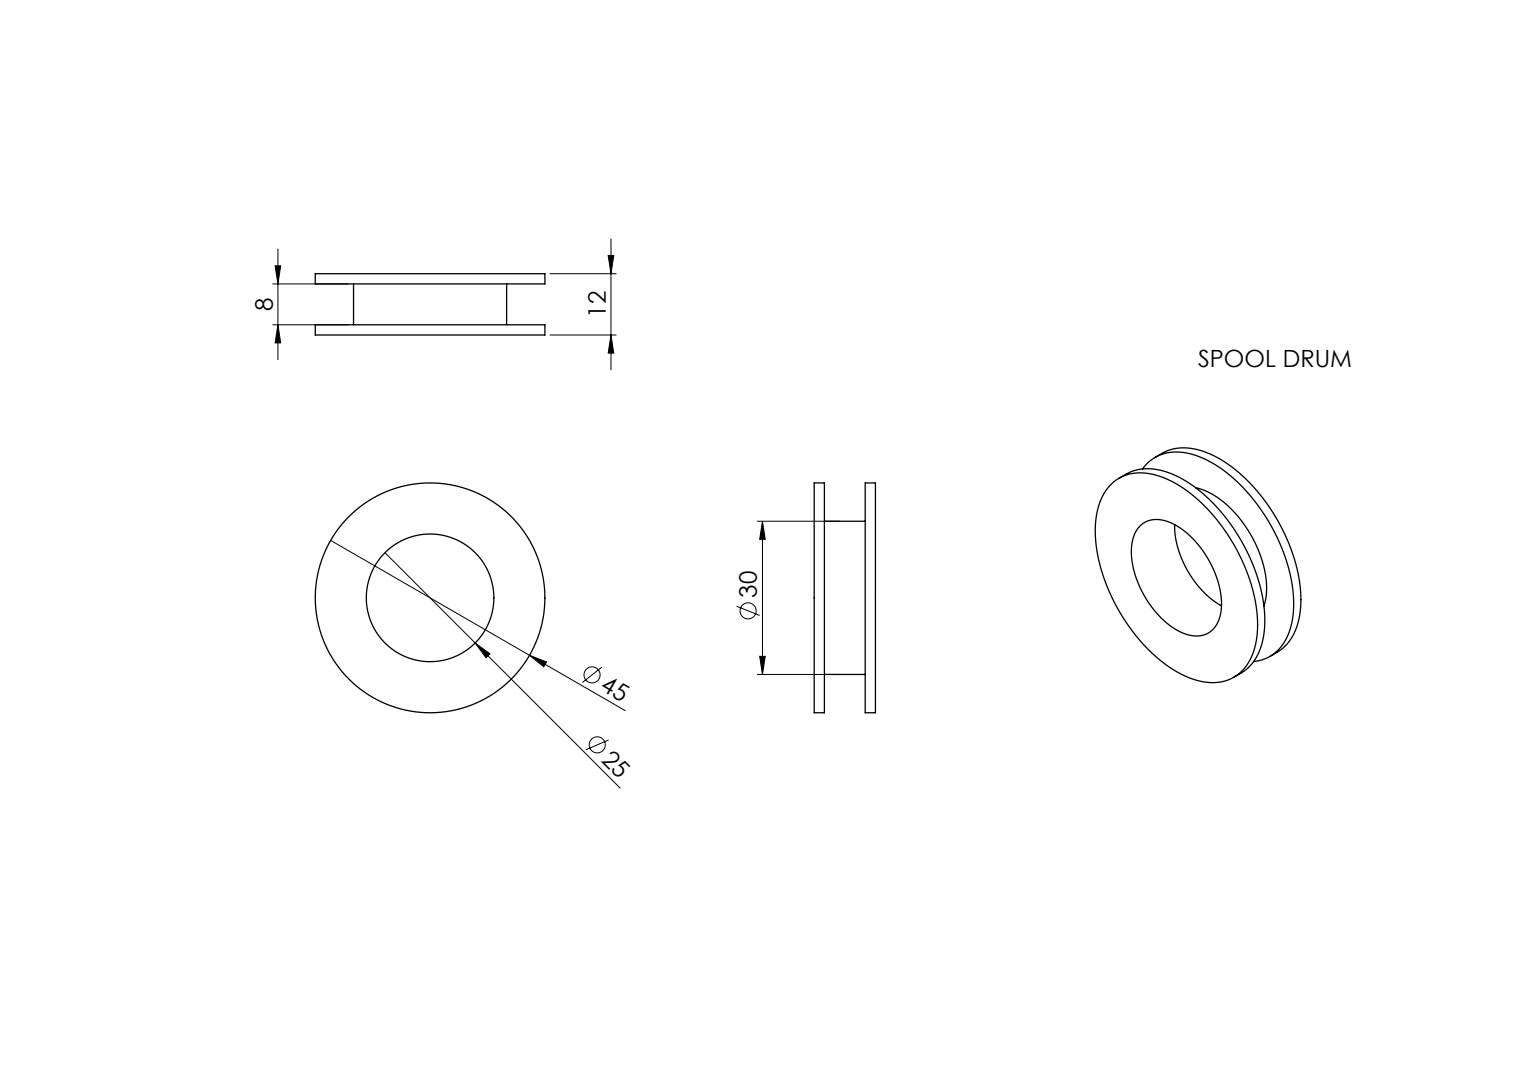
ISO-10303-21;
HEADER;
FILE_DESCRIPTION (('STEP AP214'),
    '1' );
FILE_NAME ('Spool Drum.step',
    '2026-10-23T14:45:25',
    ( '' ),
    ( '' ),
    'SwSTEP 2.0',
    'SolidWorks 2026',
    '' );
FILE_SCHEMA (( 'AUTOMOTIVE_DESIGN' ));
ENDSEC;

DATA;
#15=FACE_OUTER_BOUND ( 'NONE', #2318, .T. ) ;
#31=DIRECTION ( 'NONE',  ( -1.000000000000000000, 0.000000000000000000, 0.000000000000000000 ) ) ;
#54=VECTOR ( 'NONE', #1585, 1000.000000000000000 ) ;
#63=CARTESIAN_POINT ( 'NONE',  ( -12.50000000000000000, 0.000000000000000000, 14.00000000000000000 ) ) ;
#87=DIRECTION ( 'NONE',  ( 0.000000000000000000, 0.000000000000000000, -1.000000000000000000 ) ) ;
#91=DIRECTION ( 'NONE',  ( -0.000000000000000000, -0.000000000000000000, -1.000000000000000000 ) ) ;
#105=EDGE_CURVE ( 'NONE', #3518, #3244, #4364, .T. ) ;
#128=CARTESIAN_POINT ( 'NONE',  ( 22.50000000000000355, 2.755455298081545172E-15, 4.000000000000000000 ) ) ;
#145=LINE ( 'NONE', #1902, #3817 ) ;
#163=CIRCLE ( 'NONE', #2186, 15.00000000000000000 ) ;
#167=EDGE_CURVE ( 'NONE', #3046, #5218, #4525, .T. ) ;
#199=CARTESIAN_POINT ( 'NONE',  ( 0.000000000000000000, 0.000000000000000000, 12.00000000000000000 ) ) ;
#201=CARTESIAN_POINT ( 'NONE',  ( 0.000000000000000000, 0.000000000000000000, 14.00000000000000000 ) ) ;
#271=EDGE_LOOP ( 'NONE', ( #2578, #2682 ) ) ;
#283=CARTESIAN_POINT ( 'NONE',  ( 0.000000000000000000, 0.000000000000000000, 0.000000000000000000 ) ) ;
#310=( LENGTH_UNIT ( ) NAMED_UNIT ( * ) SI_UNIT ( .MILLI., .METRE. ) );
#312=ADVANCED_FACE ( 'NONE', ( #3377 ), #4350, .T. ) ;
#318=AXIS2_PLACEMENT_3D ( 'NONE', #1588, #1158, #4183 ) ;
#328=EDGE_CURVE ( 'NONE', #3244, #3518, #3734, .T. ) ;
#336=CARTESIAN_POINT ( 'NONE',  ( 0.000000000000000000, 0.000000000000000000, 4.000000000000000000 ) ) ;
#388=FACE_OUTER_BOUND ( 'NONE', #4673, .T. ) ;
#404=DIRECTION ( 'NONE',  ( 0.000000000000000000, 0.000000000000000000, 1.000000000000000000 ) ) ;
#409=PRODUCT_DEFINITION_SHAPE ( 'NONE', 'NONE',  #1447 ) ;
#414=AXIS2_PLACEMENT_3D ( 'NONE', #201, #3683, #2416 ) ;
#420=ORIENTED_EDGE ( 'NONE', *, *, #5372, .T. ) ;
#436=ORIENTED_EDGE ( 'NONE', *, *, #1530, .T. ) ;
#464=CARTESIAN_POINT ( 'NONE',  ( 0.000000000000000000, 0.000000000000000000, 14.00000000000000000 ) ) ;
#473=CARTESIAN_POINT ( 'NONE',  ( 0.000000000000000000, 0.000000000000000000, 2.000000000000000000 ) ) ;
#479=DIRECTION ( 'NONE',  ( 1.000000000000000000, 0.000000000000000000, 0.000000000000000000 ) ) ;
#484=DIRECTION ( 'NONE',  ( 0.000000000000000000, 0.000000000000000000, -1.000000000000000000 ) ) ;
#499=AXIS2_PLACEMENT_3D ( 'NONE', #336, #5518, #5170 ) ;
#520=AXIS2_PLACEMENT_3D ( 'NONE', #3033, #5131, #3456 ) ;
#534=VERTEX_POINT ( 'NONE', #2654 ) ;
#551=ORIENTED_EDGE ( 'NONE', *, *, #167, .T. ) ;
#567=ORIENTED_EDGE ( 'NONE', *, *, #695, .F. ) ;
#585=EDGE_CURVE ( 'NONE', #2034, #5308, #1351, .T. ) ;
#618=ORIENTED_EDGE ( 'NONE', *, *, #1353, .F. ) ;
#625=AXIS2_PLACEMENT_3D ( 'NONE', #1558, #3738, #1899 ) ;
#627=ORIENTED_EDGE ( 'NONE', *, *, #328, .T. ) ;
#647=DIRECTION ( 'NONE',  ( -0.000000000000000000, -0.000000000000000000, -1.000000000000000000 ) ) ;
#665=UNCERTAINTY_MEASURE_WITH_UNIT (LENGTH_MEASURE( 1.000000000000000082E-05 ), #5331, 'distance_accuracy_value', 'NONE');
#667=ORIENTED_EDGE ( 'NONE', *, *, #1697, .T. ) ;
#673=EDGE_LOOP ( 'NONE', ( #3634, #1342, #551, #4466 ) ) ;
#695=EDGE_CURVE ( 'NONE', #5417, #2009, #2414, .T. ) ;
#702=CARTESIAN_POINT ( 'NONE',  ( -22.50000000000000355, 0.000000000000000000, 14.00000000000000000 ) ) ;
#732=ORIENTED_EDGE ( 'NONE', *, *, #5425, .T. ) ;
#775=ADVANCED_FACE ( 'NONE', ( #4519, #5412 ), #2791, .T. ) ;
#781=DIRECTION ( 'NONE',  ( 1.000000000000000000, 0.000000000000000000, 0.000000000000000000 ) ) ;
#785=AXIS2_PLACEMENT_3D ( 'NONE', #3064, #2598, #871 ) ;
#801=DIRECTION ( 'NONE',  ( -1.000000000000000000, 0.000000000000000000, 0.000000000000000000 ) ) ;
#811=ORIENTED_EDGE ( 'NONE', *, *, #5425, .F. ) ;
#834=( NAMED_UNIT ( * ) SI_UNIT ( $, .STERADIAN. ) SOLID_ANGLE_UNIT ( ) );
#859=CIRCLE ( 'NONE', #4991, 12.50000000000000000 ) ;
#863=CIRCLE ( 'NONE', #5184, 22.50000000000000355 ) ;
#871=DIRECTION ( 'NONE',  ( -1.000000000000000000, 0.000000000000000000, 0.000000000000000000 ) ) ;
#881=CARTESIAN_POINT ( 'NONE',  ( -22.50000000000000355, 0.000000000000000000, 2.000000000000000000 ) ) ;
#886=AXIS2_PLACEMENT_3D ( 'NONE', #464, #4037, #4065 ) ;
#900=DIRECTION ( 'NONE',  ( -1.000000000000000000, 0.000000000000000000, 0.000000000000000000 ) ) ;
#934=ORIENTED_EDGE ( 'NONE', *, *, #585, .F. ) ;
#936=PLANE ( 'NONE',  #4756 ) ;
#1043=FACE_OUTER_BOUND ( 'NONE', #2938, .T. ) ;
#1046=CIRCLE ( 'NONE', #1974, 15.00000000000000000 ) ;
#1062=CARTESIAN_POINT ( 'NONE',  ( -22.50000000000000355, 0.000000000000000000, 14.00000000000000000 ) ) ;
#1091=DIRECTION ( 'NONE',  ( 0.000000000000000000, 0.000000000000000000, -1.000000000000000000 ) ) ;
#1117=VERTEX_POINT ( 'NONE', #1252 ) ;
#1119=DIRECTION ( 'NONE',  ( -1.000000000000000000, 0.000000000000000000, 0.000000000000000000 ) ) ;
#1131=DIRECTION ( 'NONE',  ( -1.000000000000000000, 0.000000000000000000, 0.000000000000000000 ) ) ;
#1158=DIRECTION ( 'NONE',  ( 0.000000000000000000, 0.000000000000000000, -1.000000000000000000 ) ) ;
#1172=AXIS2_PLACEMENT_3D ( 'NONE', #4145, #1091, #3312 ) ;
#1178=DIRECTION ( 'NONE',  ( 0.000000000000000000, 0.000000000000000000, -1.000000000000000000 ) ) ;
#1183=( NAMED_UNIT ( * ) PLANE_ANGLE_UNIT ( ) SI_UNIT ( $, .RADIAN. ) );
#1195=PRODUCT ( 'Spool Drum', 'Spool Drum', '', ( #4370 ) ) ;
#1196=CYLINDRICAL_SURFACE ( 'NONE', #785, 22.50000000000000355 ) ;
#1223=ORIENTED_EDGE ( 'NONE', *, *, #3217, .T. ) ;
#1230=DIRECTION ( 'NONE',  ( -0.000000000000000000, -0.000000000000000000, -1.000000000000000000 ) ) ;
#1247=AXIS2_PLACEMENT_3D ( 'NONE', #1760, #1390, #900 ) ;
#1252=CARTESIAN_POINT ( 'NONE',  ( -12.50000000000000000, 0.000000000000000000, 2.000000000000000000 ) ) ;
#1267=DIRECTION ( 'NONE',  ( 0.000000000000000000, 0.000000000000000000, 1.000000000000000000 ) ) ;
#1273=ORIENTED_EDGE ( 'NONE', *, *, #3459, .T. ) ;
#1276=CARTESIAN_POINT ( 'NONE',  ( 0.000000000000000000, 0.000000000000000000, 2.000000000000000000 ) ) ;
#1295=EDGE_CURVE ( 'NONE', #1815, #3046, #2550, .T. ) ;
#1301=DIRECTION ( 'NONE',  ( -1.000000000000000000, 0.000000000000000000, 0.000000000000000000 ) ) ;
#1336=AXIS2_PLACEMENT_3D ( 'NONE', #283, #2997, #5213 ) ;
#1342=ORIENTED_EDGE ( 'NONE', *, *, #4524, .F. ) ;
#1351=CIRCLE ( 'NONE', #4561, 15.00000000000000000 ) ;
#1353=EDGE_CURVE ( 'NONE', #4627, #4235, #163, .T. ) ;
#1355=DIRECTION ( 'NONE',  ( -0.000000000000000000, -0.000000000000000000, -1.000000000000000000 ) ) ;
#1367=ORIENTED_EDGE ( 'NONE', *, *, #5002, .T. ) ;
#1383=CARTESIAN_POINT ( 'NONE',  ( 0.000000000000000000, 0.000000000000000000, 12.00000000000000000 ) ) ;
#1390=DIRECTION ( 'NONE',  ( 0.000000000000000000, 0.000000000000000000, -1.000000000000000000 ) ) ;
#1414=( NAMED_UNIT ( * ) SI_UNIT ( $, .STERADIAN. ) SOLID_ANGLE_UNIT ( ) );
#1427=CARTESIAN_POINT ( 'NONE',  ( 15.00000000000000000, 1.836970198721029589E-15, 4.000000000000000000 ) ) ;
#1447=PRODUCT_DEFINITION ( 'UNKNOWN', '', #5080, #1714 ) ;
#1485=ORIENTED_EDGE ( 'NONE', *, *, #3217, .F. ) ;
#1489=ORIENTED_EDGE ( 'NONE', *, *, #1353, .T. ) ;
#1494=DIRECTION ( 'NONE',  ( 0.000000000000000000, 0.000000000000000000, 1.000000000000000000 ) ) ;
#1498=DIRECTION ( 'NONE',  ( -0.000000000000000000, -0.000000000000000000, -1.000000000000000000 ) ) ;
#1506=AXIS2_PLACEMENT_3D ( 'NONE', #4400, #1267, #4798 ) ;
#1530=EDGE_CURVE ( 'NONE', #1117, #4802, #2739, .T. ) ;
#1544=AXIS2_PLACEMENT_3D ( 'NONE', #3311, #3252, #4121 ) ;
#1552=CARTESIAN_POINT ( 'NONE',  ( -15.00000000000000000, 0.000000000000000000, 4.000000000000000000 ) ) ;
#1558=CARTESIAN_POINT ( 'NONE',  ( 0.000000000000000000, 0.000000000000000000, 2.000000000000000000 ) ) ;
#1585=DIRECTION ( 'NONE',  ( -0.000000000000000000, -0.000000000000000000, -1.000000000000000000 ) ) ;
#1588=CARTESIAN_POINT ( 'NONE',  ( 0.000000000000000000, 0.000000000000000000, 4.000000000000000000 ) ) ;
#1601=( GEOMETRIC_REPRESENTATION_CONTEXT ( 3 ) GLOBAL_UNCERTAINTY_ASSIGNED_CONTEXT ( ( #665 ) ) GLOBAL_UNIT_ASSIGNED_CONTEXT ( ( #5331, #4953, #1414 ) ) REPRESENTATION_CONTEXT ( 'NONE', 'WORKASPACE' ) );
#1610=STYLED_ITEM ( 'NONE', ( #4290 ), #4053 ) ;
#1616=EDGE_LOOP ( 'NONE', ( #3703, #2606 ) ) ;
#1625=ORIENTED_EDGE ( 'NONE', *, *, #2209, .F. ) ;
#1638=LINE ( 'NONE', #2469, #2519 ) ;
#1643=EDGE_CURVE ( 'NONE', #5218, #3309, #5673, .T. ) ;
#1694=SHAPE_REPRESENTATION_RELATIONSHIP ( 'NONE' , 'NONE' ,  #5261, #4053 ) ;
#1697=EDGE_CURVE ( 'NONE', #5417, #2170, #4021, .T. ) ;
#1714=PRODUCT_DEFINITION_CONTEXT ( 'detailed design', #3576, 'design' ) ;
#1715=AXIS2_PLACEMENT_3D ( 'NONE', #3287, #5416, #2018 ) ;
#1760=CARTESIAN_POINT ( 'NONE',  ( 0.000000000000000000, 0.000000000000000000, 4.000000000000000000 ) ) ;
#1792=COLOUR_RGB ( '',0.8941176470588234615, 0.8941176470588234615, 0.8941176470588234615 ) ;
#1801=CARTESIAN_POINT ( 'NONE',  ( 0.000000000000000000, 0.000000000000000000, 14.00000000000000000 ) ) ;
#1815=VERTEX_POINT ( 'NONE', #4230 ) ;
#1867=EDGE_LOOP ( 'NONE', ( #436, #3178 ) ) ;
#1891=ORIENTED_EDGE ( 'NONE', *, *, #5677, .T. ) ;
#1899=DIRECTION ( 'NONE',  ( 1.000000000000000000, 0.000000000000000000, 0.000000000000000000 ) ) ;
#1902=CARTESIAN_POINT ( 'NONE',  ( -12.50000000000000000, 0.000000000000000000, 14.00000000000000000 ) ) ;
#1919=ORIENTED_EDGE ( 'NONE', *, *, #1643, .F. ) ;
#1932=DIRECTION ( 'NONE',  ( 0.000000000000000000, 0.000000000000000000, 1.000000000000000000 ) ) ;
#1943=ADVANCED_FACE ( 'NONE', ( #388 ), #4880, .T. ) ;
#1954=ADVANCED_FACE ( 'NONE', ( #5659, #3474 ), #936, .F. ) ;
#1964=DIRECTION ( 'NONE',  ( 1.000000000000000000, 0.000000000000000000, 0.000000000000000000 ) ) ;
#1974=AXIS2_PLACEMENT_3D ( 'NONE', #1383, #4375, #4828 ) ;
#1988=UNCERTAINTY_MEASURE_WITH_UNIT (LENGTH_MEASURE( 1.000000000000000082E-05 ), #3797, 'distance_accuracy_value', 'NONE');
#2000=EDGE_LOOP ( 'NONE', ( #4635, #4038 ) ) ;
#2009=VERTEX_POINT ( 'NONE', #881 ) ;
#2018=DIRECTION ( 'NONE',  ( 1.000000000000000000, 0.000000000000000000, 0.000000000000000000 ) ) ;
#2034=VERTEX_POINT ( 'NONE', #1427 ) ;
#2072=SURFACE_STYLE_USAGE ( .BOTH. , #2963 ) ;
#2098=( NAMED_UNIT ( * ) PLANE_ANGLE_UNIT ( ) SI_UNIT ( $, .RADIAN. ) );
#2103=ORIENTED_EDGE ( 'NONE', *, *, #167, .F. ) ;
#2149=DIRECTION ( 'NONE',  ( -0.000000000000000000, -0.000000000000000000, -1.000000000000000000 ) ) ;
#2170=VERTEX_POINT ( 'NONE', #128 ) ;
#2186=AXIS2_PLACEMENT_3D ( 'NONE', #4834, #484, #1301 ) ;
#2209=EDGE_CURVE ( 'NONE', #5308, #2034, #2251, .T. ) ;
#2230=EDGE_LOOP ( 'NONE', ( #667, #1223, #4104, #567 ) ) ;
#2251=CIRCLE ( 'NONE', #318, 15.00000000000000000 ) ;
#2265=ADVANCED_FACE ( 'NONE', ( #2481 ), #3319, .F. ) ;
#2271=AXIS2_PLACEMENT_3D ( 'NONE', #5270, #3087, #2741 ) ;
#2304=LINE ( 'NONE', #5390, #54 ) ;
#2318=EDGE_LOOP ( 'NONE', ( #4210, #3063 ) ) ;
#2331=ORIENTED_EDGE ( 'NONE', *, *, #1295, .F. ) ;
#2383=ORIENTED_EDGE ( 'NONE', *, *, #4995, .F. ) ;
#2399=CYLINDRICAL_SURFACE ( 'NONE', #4461, 15.00000000000000000 ) ;
#2410=( GEOMETRIC_REPRESENTATION_CONTEXT ( 3 ) GLOBAL_UNCERTAINTY_ASSIGNED_CONTEXT ( ( #1988 ) ) GLOBAL_UNIT_ASSIGNED_CONTEXT ( ( #3797, #2098, #3883 ) ) REPRESENTATION_CONTEXT ( 'NONE', 'WORKASPACE' ) );
#2414=LINE ( 'NONE', #1062, #3380 ) ;
#2416=DIRECTION ( 'NONE',  ( -1.000000000000000000, 0.000000000000000000, 0.000000000000000000 ) ) ;
#2438=FACE_BOUND ( 'NONE', #3207, .T. ) ;
#2451=ORIENTED_EDGE ( 'NONE', *, *, #1643, .T. ) ;
#2469=CARTESIAN_POINT ( 'NONE',  ( 12.50000000000000000, 1.530808498934191521E-15, 14.00000000000000000 ) ) ;
#2473=EDGE_CURVE ( 'NONE', #534, #2009, #4820, .T. ) ;
#2481=FACE_OUTER_BOUND ( 'NONE', #2838, .T. ) ;
#2519=VECTOR ( 'NONE', #1230, 1000.000000000000000 ) ;
#2550=CIRCLE ( 'NONE', #2271, 22.50000000000000355 ) ;
#2578=ORIENTED_EDGE ( 'NONE', *, *, #1697, .F. ) ;
#2598=DIRECTION ( 'NONE',  ( -0.000000000000000000, -0.000000000000000000, -1.000000000000000000 ) ) ;
#2606=ORIENTED_EDGE ( 'NONE', *, *, #2473, .F. ) ;
#2621=AXIS2_PLACEMENT_3D ( 'NONE', #1276, #4297, #479 ) ;
#2649=LINE ( 'NONE', #3994, #3993 ) ;
#2654=CARTESIAN_POINT ( 'NONE',  ( 22.50000000000000355, 2.755455298081545172E-15, 2.000000000000000000 ) ) ;
#2682=ORIENTED_EDGE ( 'NONE', *, *, #3286, .F. ) ;
#2721=EDGE_CURVE ( 'NONE', #4627, #5308, #2967, .T. ) ;
#2739=CIRCLE ( 'NONE', #625, 12.50000000000000000 ) ;
#2741=DIRECTION ( 'NONE',  ( 1.000000000000000000, 0.000000000000000000, 0.000000000000000000 ) ) ;
#2764=ORIENTED_EDGE ( 'NONE', *, *, #105, .T. ) ;
#2789=DIRECTION ( 'NONE',  ( 0.000000000000000000, 0.000000000000000000, -1.000000000000000000 ) ) ;
#2791=PLANE ( 'NONE',  #1172 ) ;
#2793=ADVANCED_FACE ( 'NONE', ( #1043 ), #2399, .T. ) ;
#2838=EDGE_LOOP ( 'NONE', ( #811, #2764, #1891, #5334 ) ) ;
#2853=CYLINDRICAL_SURFACE ( 'NONE', #414, 22.50000000000000355 ) ;
#2872=CARTESIAN_POINT ( 'NONE',  ( 0.000000000000000000, 0.000000000000000000, 12.00000000000000000 ) ) ;
#2882=DIRECTION ( 'NONE',  ( -1.000000000000000000, 0.000000000000000000, 0.000000000000000000 ) ) ;
#2901=CYLINDRICAL_SURFACE ( 'NONE', #3904, 15.00000000000000000 ) ;
#2938=EDGE_LOOP ( 'NONE', ( #4203, #3297, #3304, #934 ) ) ;
#2955=AXIS2_PLACEMENT_3D ( 'NONE', #4976, #1932, #5504 ) ;
#2957=CARTESIAN_POINT ( 'NONE',  ( -22.50000000000000355, 0.000000000000000000, 4.000000000000000000 ) ) ;
#2963=SURFACE_SIDE_STYLE ('',( #5152 ) ) ;
#2967=LINE ( 'NONE', #4715, #5472 ) ;
#2997=DIRECTION ( 'NONE',  ( 0.000000000000000000, 0.000000000000000000, 1.000000000000000000 ) ) ;
#3006=VECTOR ( 'NONE', #4151, 1000.000000000000000 ) ;
#3033=CARTESIAN_POINT ( 'NONE',  ( 0.000000000000000000, 0.000000000000000000, 14.00000000000000000 ) ) ;
#3046=VERTEX_POINT ( 'NONE', #5137 ) ;
#3063=ORIENTED_EDGE ( 'NONE', *, *, #1295, .T. ) ;
#3064=CARTESIAN_POINT ( 'NONE',  ( 0.000000000000000000, 0.000000000000000000, 14.00000000000000000 ) ) ;
#3083=PLANE ( 'NONE',  #1506 ) ;
#3087=DIRECTION ( 'NONE',  ( 0.000000000000000000, 0.000000000000000000, 1.000000000000000000 ) ) ;
#3138=ADVANCED_FACE ( 'NONE', ( #3384 ), #1196, .T. ) ;
#3171=STYLED_ITEM('',(#5716),#4501);
#3178=ORIENTED_EDGE ( 'NONE', *, *, #4247, .T. ) ;
#3184=ORIENTED_EDGE ( 'NONE', *, *, #2209, .T. ) ;
#3207=EDGE_LOOP ( 'NONE', ( #3184, #4385 ) ) ;
#3217=EDGE_CURVE ( 'NONE', #2170, #534, #5332, .T. ) ;
#3244=VERTEX_POINT ( 'NONE', #63 ) ;
#3252=DIRECTION ( 'NONE',  ( 0.000000000000000000, 0.000000000000000000, -1.000000000000000000 ) ) ;
#3254=FACE_OUTER_BOUND ( 'NONE', #673, .T. ) ;
#3285=AXIS2_PLACEMENT_3D ( 'NONE', #199, #2789, #1119 ) ;
#3286=EDGE_CURVE ( 'NONE', #2170, #5417, #4648, .T. ) ;
#3287=CARTESIAN_POINT ( 'NONE',  ( 0.000000000000000000, 0.000000000000000000, 2.000000000000000000 ) ) ;
#3297=ORIENTED_EDGE ( 'NONE', *, *, #4995, .T. ) ;
#3304=ORIENTED_EDGE ( 'NONE', *, *, #2721, .T. ) ;
#3309=VERTEX_POINT ( 'NONE', #4926 ) ;
#3311=CARTESIAN_POINT ( 'NONE',  ( 0.000000000000000000, 0.000000000000000000, 4.000000000000000000 ) ) ;
#3312=DIRECTION ( 'NONE',  ( -1.000000000000000000, 0.000000000000000000, -0.000000000000000000 ) ) ;
#3314=DIRECTION ( 'NONE',  ( -0.000000000000000000, -0.000000000000000000, -1.000000000000000000 ) ) ;
#3319=CYLINDRICAL_SURFACE ( 'NONE', #3359, 12.50000000000000000 ) ;
#3334=ADVANCED_FACE ( 'NONE', ( #3546 ), #4870, .F. ) ;
#3359=AXIS2_PLACEMENT_3D ( 'NONE', #5444, #1498, #2882 ) ;
#3360=( GEOMETRIC_REPRESENTATION_CONTEXT ( 3 ) GLOBAL_UNCERTAINTY_ASSIGNED_CONTEXT ( ( #4179 ) ) GLOBAL_UNIT_ASSIGNED_CONTEXT ( ( #310, #1183, #834 ) ) REPRESENTATION_CONTEXT ( 'NONE', 'WORKASPACE' ) );
#3368=VECTOR ( 'NONE', #91, 1000.000000000000000 ) ;
#3371=CIRCLE ( 'NONE', #1715, 22.50000000000000355 ) ;
#3377=FACE_OUTER_BOUND ( 'NONE', #2230, .T. ) ;
#3380=VECTOR ( 'NONE', #4175, 1000.000000000000000 ) ;
#3384=FACE_OUTER_BOUND ( 'NONE', #4966, .T. ) ;
#3403=CARTESIAN_POINT ( 'NONE',  ( 0.000000000000000000, 0.000000000000000000, 14.00000000000000000 ) ) ;
#3432=EDGE_LOOP ( 'NONE', ( #2451, #420 ) ) ;
#3456=DIRECTION ( 'NONE',  ( -1.000000000000000000, 0.000000000000000000, 0.000000000000000000 ) ) ;
#3459=EDGE_CURVE ( 'NONE', #1815, #3309, #2304, .T. ) ;
#3474=FACE_BOUND ( 'NONE', #1867, .T. ) ;
#3518=VERTEX_POINT ( 'NONE', #5440 ) ;
#3522=FACE_BOUND ( 'NONE', #2000, .T. ) ;
#3533=AXIS2_PLACEMENT_3D ( 'NONE', #4735, #1178, #801 ) ;
#3546=FACE_OUTER_BOUND ( 'NONE', #4190, .T. ) ;
#3565=AXIS2_PLACEMENT_3D ( 'NONE', #1801, #2149, #3903 ) ;
#3576=APPLICATION_CONTEXT ( 'automotive_design' ) ;
#3612=ORIENTED_EDGE ( 'NONE', *, *, #1530, .F. ) ;
#3634=ORIENTED_EDGE ( 'NONE', *, *, #3459, .F. ) ;
#3638=EDGE_CURVE ( 'NONE', #2009, #534, #3371, .T. ) ;
#3683=DIRECTION ( 'NONE',  ( -0.000000000000000000, -0.000000000000000000, -1.000000000000000000 ) ) ;
#3684=CARTESIAN_POINT ( 'NONE',  ( 0.000000000000000000, 0.000000000000000000, 14.00000000000000000 ) ) ;
#3703=ORIENTED_EDGE ( 'NONE', *, *, #3638, .F. ) ;
#3734=CIRCLE ( 'NONE', #5023, 12.50000000000000000 ) ;
#3738=DIRECTION ( 'NONE',  ( 0.000000000000000000, 0.000000000000000000, 1.000000000000000000 ) ) ;
#3751=CARTESIAN_POINT ( 'NONE',  ( 15.00000000000000000, 1.836970198721029589E-15, 12.00000000000000000 ) ) ;
#3760=APPLICATION_CONTEXT ( 'automotive_design' ) ;
#3797=( LENGTH_UNIT ( ) NAMED_UNIT ( * ) SI_UNIT ( .MILLI., .METRE. ) );
#3817=VECTOR ( 'NONE', #3314, 1000.000000000000000 ) ;
#3883=( NAMED_UNIT ( * ) SI_UNIT ( $, .STERADIAN. ) SOLID_ANGLE_UNIT ( ) );
#3903=DIRECTION ( 'NONE',  ( -1.000000000000000000, 0.000000000000000000, 0.000000000000000000 ) ) ;
#3904=AXIS2_PLACEMENT_3D ( 'NONE', #2872, #4252, #4624 ) ;
#3976=ORIENTED_EDGE ( 'NONE', *, *, #3286, .T. ) ;
#3993=VECTOR ( 'NONE', #1355, 1000.000000000000000 ) ;
#3994=CARTESIAN_POINT ( 'NONE',  ( 15.00000000000000000, 1.836970198721029589E-15, 12.00000000000000000 ) ) ;
#4021=CIRCLE ( 'NONE', #1544, 22.50000000000000355 ) ;
#4036=DIRECTION ( 'NONE',  ( 1.000000000000000000, 0.000000000000000000, 0.000000000000000000 ) ) ;
#4037=DIRECTION ( 'NONE',  ( -0.000000000000000000, -0.000000000000000000, -1.000000000000000000 ) ) ;
#4038=ORIENTED_EDGE ( 'NONE', *, *, #105, .F. ) ;
#4053=ADVANCED_BREP_SHAPE_REPRESENTATION ( '', ( #4501, #1336 ), #3360 ) ;
#4065=DIRECTION ( 'NONE',  ( -1.000000000000000000, 0.000000000000000000, 0.000000000000000000 ) ) ;
#4067=EDGE_LOOP ( 'NONE', ( #618, #2383 ) ) ;
#4104=ORIENTED_EDGE ( 'NONE', *, *, #2473, .T. ) ;
#4121=DIRECTION ( 'NONE',  ( -1.000000000000000000, 0.000000000000000000, 0.000000000000000000 ) ) ;
#4139=CARTESIAN_POINT ( 'NONE',  ( -22.50000000000000355, 0.000000000000000000, 12.00000000000000000 ) ) ;
#4145=CARTESIAN_POINT ( 'NONE',  ( 0.000000000000000000, 0.000000000000000000, 12.00000000000000000 ) ) ;
#4151=DIRECTION ( 'NONE',  ( -0.000000000000000000, -0.000000000000000000, -1.000000000000000000 ) ) ;
#4157=DIRECTION ( 'NONE',  ( 0.000000000000000000, 0.000000000000000000, 1.000000000000000000 ) ) ;
#4175=DIRECTION ( 'NONE',  ( -0.000000000000000000, -0.000000000000000000, -1.000000000000000000 ) ) ;
#4179=UNCERTAINTY_MEASURE_WITH_UNIT (LENGTH_MEASURE( 1.000000000000000082E-05 ), #310, 'distance_accuracy_value', 'NONE');
#4183=DIRECTION ( 'NONE',  ( -1.000000000000000000, 0.000000000000000000, 0.000000000000000000 ) ) ;
#4190=EDGE_LOOP ( 'NONE', ( #627, #732, #3612, #4219 ) ) ;
#4200=FACE_OUTER_BOUND ( 'NONE', #271, .T. ) ;
#4203=ORIENTED_EDGE ( 'NONE', *, *, #5002, .F. ) ;
#4210=ORIENTED_EDGE ( 'NONE', *, *, #4524, .T. ) ;
#4216=CARTESIAN_POINT ( 'NONE',  ( 0.000000000000000000, 0.000000000000000000, 2.000000000000000000 ) ) ;
#4219=ORIENTED_EDGE ( 'NONE', *, *, #5677, .F. ) ;
#4230=CARTESIAN_POINT ( 'NONE',  ( 22.50000000000000355, 2.755455298081545172E-15, 14.00000000000000000 ) ) ;
#4235=VERTEX_POINT ( 'NONE', #3751 ) ;
#4247=EDGE_CURVE ( 'NONE', #4802, #1117, #859, .T. ) ;
#4252=DIRECTION ( 'NONE',  ( -0.000000000000000000, -0.000000000000000000, -1.000000000000000000 ) ) ;
#4259=FILL_AREA_STYLE ('',( #4711 ) ) ;
#4281=ORIENTED_EDGE ( 'NONE', *, *, #2721, .F. ) ;
#4290=PRESENTATION_STYLE_ASSIGNMENT (( #2072 ) ) ;
#4297=DIRECTION ( 'NONE',  ( 0.000000000000000000, 0.000000000000000000, 1.000000000000000000 ) ) ;
#4348=DIRECTION ( 'NONE',  ( -0.000000000000000000, -0.000000000000000000, -1.000000000000000000 ) ) ;
#4350=CYLINDRICAL_SURFACE ( 'NONE', #520, 22.50000000000000355 ) ;
#4364=CIRCLE ( 'NONE', #2955, 12.50000000000000000 ) ;
#4370=PRODUCT_CONTEXT ( 'NONE', #3760, 'mechanical' ) ;
#4375=DIRECTION ( 'NONE',  ( 0.000000000000000000, 0.000000000000000000, -1.000000000000000000 ) ) ;
#4385=ORIENTED_EDGE ( 'NONE', *, *, #585, .T. ) ;
#4400=CARTESIAN_POINT ( 'NONE',  ( 0.000000000000000000, 0.000000000000000000, 14.00000000000000000 ) ) ;
#4415=CARTESIAN_POINT ( 'NONE',  ( 12.50000000000000000, 1.530808498934191521E-15, 2.000000000000000000 ) ) ;
#4461=AXIS2_PLACEMENT_3D ( 'NONE', #5018, #647, #1131 ) ;
#4466=ORIENTED_EDGE ( 'NONE', *, *, #5372, .F. ) ;
#4501=MANIFOLD_SOLID_BREP ( 'Cut-Extrude-Thin1', #5210 ) ;
#4519=FACE_BOUND ( 'NONE', #4067, .T. ) ;
#4524=EDGE_CURVE ( 'NONE', #3046, #1815, #863, .T. ) ;
#4525=LINE ( 'NONE', #702, #3006 ) ;
#4561=AXIS2_PLACEMENT_3D ( 'NONE', #5301, #87, #31 ) ;
#4614=ORIENTED_EDGE ( 'NONE', *, *, #3638, .T. ) ;
#4624=DIRECTION ( 'NONE',  ( -1.000000000000000000, 0.000000000000000000, 0.000000000000000000 ) ) ;
#4627=VERTEX_POINT ( 'NONE', #5284 ) ;
#4635=ORIENTED_EDGE ( 'NONE', *, *, #328, .F. ) ;
#4648=CIRCLE ( 'NONE', #1247, 22.50000000000000355 ) ;
#4654=PLANE ( 'NONE',  #499 ) ;
#4664=EDGE_LOOP ( 'NONE', ( #1489, #1367, #1625, #4281 ) ) ;
#4673=EDGE_LOOP ( 'NONE', ( #1485, #3976, #5611, #4614 ) ) ;
#4711=FILL_AREA_STYLE_COLOUR ( '', #1792 ) ;
#4715=CARTESIAN_POINT ( 'NONE',  ( -15.00000000000000000, 0.000000000000000000, 12.00000000000000000 ) ) ;
#4735=CARTESIAN_POINT ( 'NONE',  ( 0.000000000000000000, 0.000000000000000000, 12.00000000000000000 ) ) ;
#4756=AXIS2_PLACEMENT_3D ( 'NONE', #473, #5234, #5260 ) ;
#4798=DIRECTION ( 'NONE',  ( 1.000000000000000000, 0.000000000000000000, -0.000000000000000000 ) ) ;
#4802=VERTEX_POINT ( 'NONE', #4415 ) ;
#4820=CIRCLE ( 'NONE', #2621, 22.50000000000000355 ) ;
#4828=DIRECTION ( 'NONE',  ( -1.000000000000000000, 0.000000000000000000, 0.000000000000000000 ) ) ;
#4832=ADVANCED_FACE ( 'NONE', ( #15, #3522 ), #3083, .T. ) ;
#4834=CARTESIAN_POINT ( 'NONE',  ( 0.000000000000000000, 0.000000000000000000, 12.00000000000000000 ) ) ;
#4841=CARTESIAN_POINT ( 'NONE',  ( 22.50000000000000355, 2.755455298081545172E-15, 14.00000000000000000 ) ) ;
#4870=CYLINDRICAL_SURFACE ( 'NONE', #886, 12.50000000000000000 ) ;
#4880=CYLINDRICAL_SURFACE ( 'NONE', #3565, 22.50000000000000355 ) ;
#4893=MECHANICAL_DESIGN_GEOMETRIC_PRESENTATION_REPRESENTATION('',(#1610),#2410);
#4915=CIRCLE ( 'NONE', #3533, 22.50000000000000355 ) ;
#4926=CARTESIAN_POINT ( 'NONE',  ( 22.50000000000000355, 2.755455298081545172E-15, 12.00000000000000000 ) ) ;
#4953=( NAMED_UNIT ( * ) PLANE_ANGLE_UNIT ( ) SI_UNIT ( $, .RADIAN. ) );
#4966=EDGE_LOOP ( 'NONE', ( #2331, #1273, #1919, #2103 ) ) ;
#4976=CARTESIAN_POINT ( 'NONE',  ( 0.000000000000000000, 0.000000000000000000, 14.00000000000000000 ) ) ;
#4991=AXIS2_PLACEMENT_3D ( 'NONE', #4216, #4157, #1964 ) ;
#4995=EDGE_CURVE ( 'NONE', #4235, #4627, #1046, .T. ) ;
#5002=EDGE_CURVE ( 'NONE', #4235, #2034, #2649, .T. ) ;
#5018=CARTESIAN_POINT ( 'NONE',  ( 0.000000000000000000, 0.000000000000000000, 12.00000000000000000 ) ) ;
#5023=AXIS2_PLACEMENT_3D ( 'NONE', #3403, #404, #781 ) ;
#5056=FACE_OUTER_BOUND ( 'NONE', #4664, .T. ) ;
#5080=PRODUCT_DEFINITION_FORMATION_WITH_SPECIFIED_SOURCE ( 'ANY', '', #1195, .NOT_KNOWN. ) ;
#5094=MECHANICAL_DESIGN_GEOMETRIC_PRESENTATION_REPRESENTATION('',(#3171),#1601);
#5131=DIRECTION ( 'NONE',  ( -0.000000000000000000, -0.000000000000000000, -1.000000000000000000 ) ) ;
#5137=CARTESIAN_POINT ( 'NONE',  ( -22.50000000000000355, 0.000000000000000000, 14.00000000000000000 ) ) ;
#5152=SURFACE_STYLE_FILL_AREA ( #4259 ) ;
#5170=DIRECTION ( 'NONE',  ( -1.000000000000000000, 0.000000000000000000, -0.000000000000000000 ) ) ;
#5184=AXIS2_PLACEMENT_3D ( 'NONE', #3684, #1494, #4036 ) ;
#5210=CLOSED_SHELL ( 'NONE', ( #5356, #3334, #312, #3138, #5627, #4832, #1954, #1943, #2265, #775, #5364, #2793 ) ) ;
#5213=DIRECTION ( 'NONE',  ( 1.000000000000000000, 0.000000000000000000, 0.000000000000000000 ) ) ;
#5218=VERTEX_POINT ( 'NONE', #4139 ) ;
#5234=DIRECTION ( 'NONE',  ( 0.000000000000000000, 0.000000000000000000, 1.000000000000000000 ) ) ;
#5260=DIRECTION ( 'NONE',  ( 1.000000000000000000, 0.000000000000000000, -0.000000000000000000 ) ) ;
#5261=SHAPE_REPRESENTATION ( 'Spool Drum', ( #1336 ), #3360 ) ;
#5270=CARTESIAN_POINT ( 'NONE',  ( 0.000000000000000000, 0.000000000000000000, 14.00000000000000000 ) ) ;
#5284=CARTESIAN_POINT ( 'NONE',  ( -15.00000000000000000, 0.000000000000000000, 12.00000000000000000 ) ) ;
#5291=SHAPE_DEFINITION_REPRESENTATION ( #409, #5261 ) ;
#5301=CARTESIAN_POINT ( 'NONE',  ( 0.000000000000000000, 0.000000000000000000, 4.000000000000000000 ) ) ;
#5308=VERTEX_POINT ( 'NONE', #1552 ) ;
#5331=( LENGTH_UNIT ( ) NAMED_UNIT ( * ) SI_UNIT ( .MILLI., .METRE. ) );
#5332=LINE ( 'NONE', #4841, #3368 ) ;
#5334=ORIENTED_EDGE ( 'NONE', *, *, #4247, .F. ) ;
#5356=ADVANCED_FACE ( 'NONE', ( #5056 ), #2901, .T. ) ;
#5364=ADVANCED_FACE ( 'NONE', ( #2438, #4200 ), #4654, .F. ) ;
#5372=EDGE_CURVE ( 'NONE', #3309, #5218, #4915, .T. ) ;
#5390=CARTESIAN_POINT ( 'NONE',  ( 22.50000000000000355, 2.755455298081545172E-15, 14.00000000000000000 ) ) ;
#5412=FACE_OUTER_BOUND ( 'NONE', #3432, .T. ) ;
#5416=DIRECTION ( 'NONE',  ( 0.000000000000000000, 0.000000000000000000, 1.000000000000000000 ) ) ;
#5417=VERTEX_POINT ( 'NONE', #2957 ) ;
#5425=EDGE_CURVE ( 'NONE', #3518, #4802, #1638, .T. ) ;
#5440=CARTESIAN_POINT ( 'NONE',  ( 12.50000000000000000, 1.530808498934191521E-15, 14.00000000000000000 ) ) ;
#5444=CARTESIAN_POINT ( 'NONE',  ( 0.000000000000000000, 0.000000000000000000, 14.00000000000000000 ) ) ;
#5472=VECTOR ( 'NONE', #4348, 1000.000000000000000 ) ;
#5504=DIRECTION ( 'NONE',  ( 1.000000000000000000, 0.000000000000000000, 0.000000000000000000 ) ) ;
#5518=DIRECTION ( 'NONE',  ( 0.000000000000000000, 0.000000000000000000, -1.000000000000000000 ) ) ;
#5611=ORIENTED_EDGE ( 'NONE', *, *, #695, .T. ) ;
#5627=ADVANCED_FACE ( 'NONE', ( #3254 ), #2853, .T. ) ;
#5659=FACE_OUTER_BOUND ( 'NONE', #1616, .T. ) ;
#5673=CIRCLE ( 'NONE', #3285, 22.50000000000000355 ) ;
#5677=EDGE_CURVE ( 'NONE', #3244, #1117, #145, .T. ) ;
#5710=COLOUR_RGB('Sky Blue',0.24,0.69,0.87);
#5711=FILL_AREA_STYLE_COLOUR('',#5710);
#5712=FILL_AREA_STYLE('',(#5711));
#5713=SURFACE_STYLE_FILL_AREA(#5712);
#5714=SURFACE_SIDE_STYLE('',(#5713));
#5715=SURFACE_STYLE_USAGE(.BOTH.,#5714);
#5716=PRESENTATION_STYLE_ASSIGNMENT((#5715));
ENDSEC;
END-ISO-10303-21;
